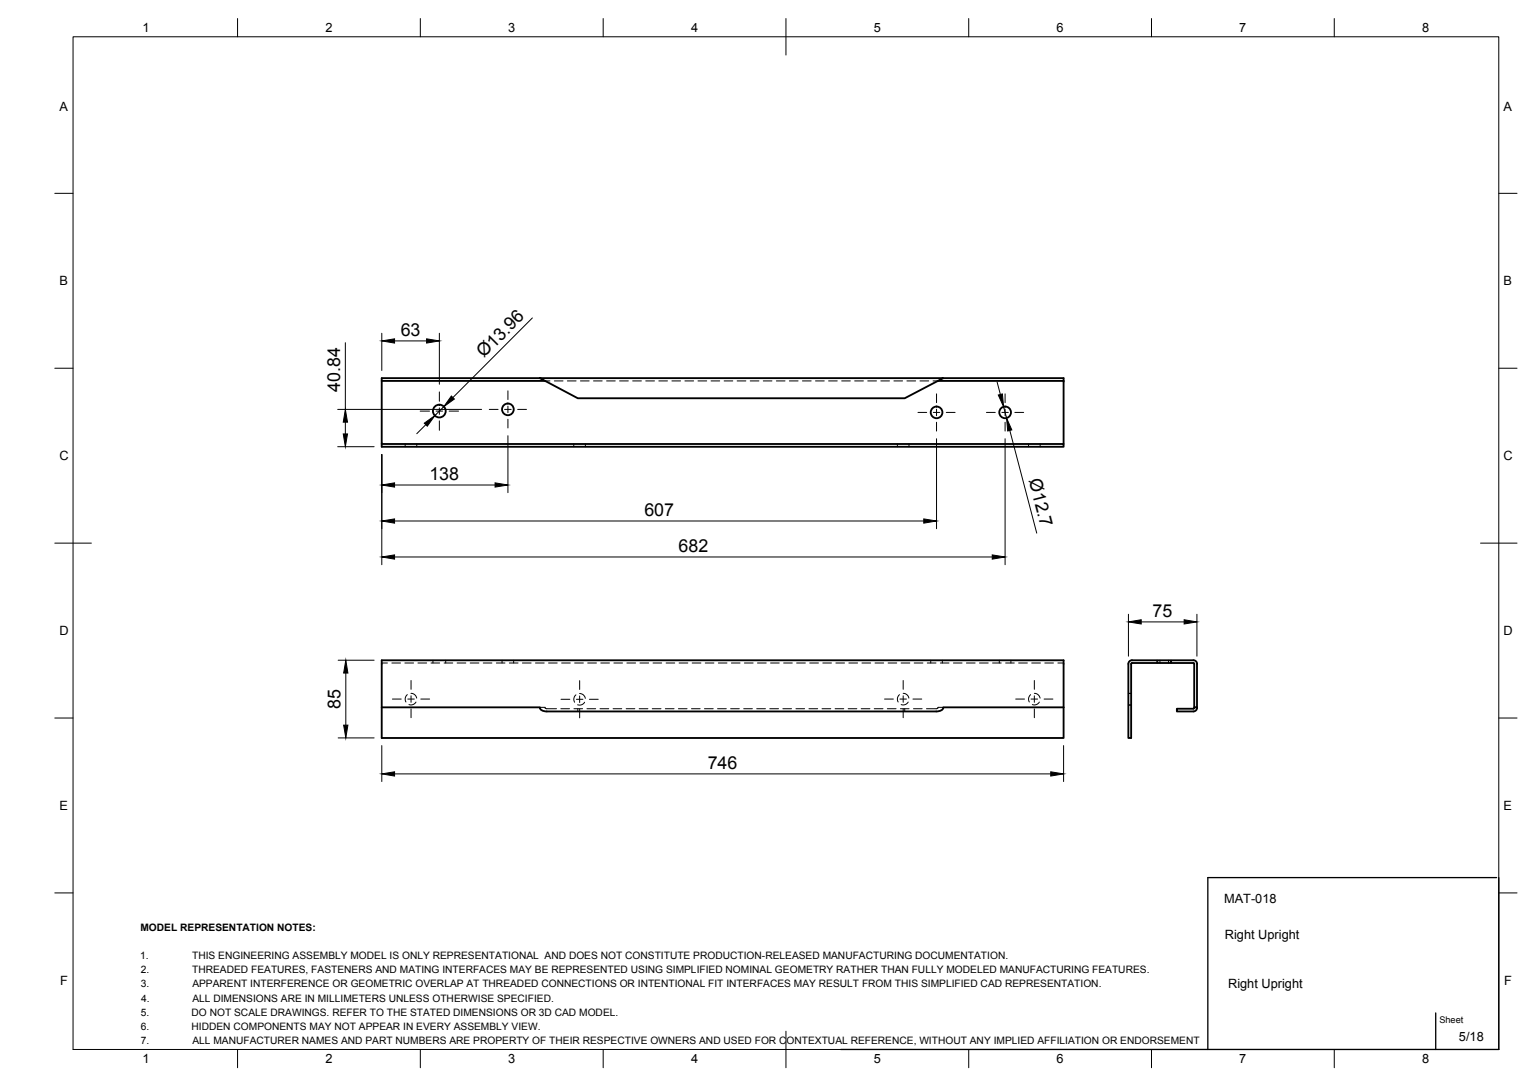
ISO-10303-21;
HEADER;
/* Generated by software containing ST-Developer
 * from STEP Tools, Inc. (www.steptools.com) 
 */

FILE_DESCRIPTION(
/* description */ ('STEP AP214'),
/* implementation_level */ '2;1');

FILE_NAME(
/* name */ 'Right Upright.step',
/* time_stamp */ '2026-11-14T06:16:09-08:00',
/* author */ (''),
/* organization */ (''),
/* preprocessor_version */ 'ST-DEVELOPER v20.2',
/* originating_system */ 'Autodesk Translation Framework v15.17.0.0',
/* authorisation */ '');

FILE_SCHEMA (('AUTOMOTIVE_DESIGN { 1 0 10303 214 3 1 1 }'));
ENDSEC;

DATA;
#10=MECHANICAL_DESIGN_GEOMETRIC_PRESENTATION_REPRESENTATION('',(#349),#18006);
#268=ELLIPSE('',#10059,8.64513309637285,4.00000000000059);
#269=ELLIPSE('',#10060,8.53586336233429,3.99999999999978);
#270=ELLIPSE('',#10073,2.16128327409315,1.00000000000008);
#271=ELLIPSE('',#10074,2.1339658405822,0.999999999999361);
#317=SHAPE_REPRESENTATION_RELATIONSHIP('SRR','None',#18073,#333);
#333=ADVANCED_BREP_SHAPE_REPRESENTATION('',(#365),#17990);
#349=STYLED_ITEM('',(#18170),#365);
#365=MANIFOLD_SOLID_BREP('Body1',#9558);
#417=FACE_BOUND('',#1638,.T.);
#418=FACE_BOUND('',#1639,.T.);
#419=FACE_BOUND('',#1640,.T.);
#420=FACE_BOUND('',#1641,.T.);
#421=FACE_BOUND('',#1644,.T.);
#422=FACE_BOUND('',#1645,.T.);
#423=FACE_BOUND('',#1646,.T.);
#424=FACE_BOUND('',#1647,.T.);
#425=FACE_BOUND('',#1650,.T.);
#426=FACE_BOUND('',#1651,.T.);
#427=FACE_BOUND('',#1652,.T.);
#428=FACE_BOUND('',#1653,.T.);
#429=FACE_BOUND('',#1656,.T.);
#430=FACE_BOUND('',#1657,.T.);
#431=FACE_BOUND('',#1658,.T.);
#432=FACE_BOUND('',#1659,.T.);
#614=PLANE('',#10038);
#615=PLANE('',#10039);
#616=PLANE('',#10042);
#617=PLANE('',#10043);
#618=PLANE('',#10046);
#619=PLANE('',#10047);
#620=PLANE('',#10050);
#621=PLANE('',#10051);
#622=PLANE('',#10054);
#623=PLANE('',#10055);
#624=PLANE('',#10056);
#625=PLANE('',#10057);
#626=PLANE('',#10061);
#627=PLANE('',#10063);
#628=PLANE('',#10065);
#629=PLANE('',#10066);
#630=PLANE('',#10067);
#631=PLANE('',#10069);
#632=PLANE('',#10071);
#633=PLANE('',#10075);
#634=PLANE('',#10076);
#635=PLANE('',#10077);
#636=PLANE('',#10078);
#637=PLANE('',#10079);
#1000=FACE_OUTER_BOUND('',#1614,.T.);
#1001=FACE_OUTER_BOUND('',#1615,.T.);
#1002=FACE_OUTER_BOUND('',#1616,.T.);
#1003=FACE_OUTER_BOUND('',#1617,.T.);
#1004=FACE_OUTER_BOUND('',#1618,.T.);
#1005=FACE_OUTER_BOUND('',#1619,.T.);
#1006=FACE_OUTER_BOUND('',#1620,.T.);
#1007=FACE_OUTER_BOUND('',#1621,.T.);
#1008=FACE_OUTER_BOUND('',#1622,.T.);
#1009=FACE_OUTER_BOUND('',#1623,.T.);
#1010=FACE_OUTER_BOUND('',#1624,.T.);
#1011=FACE_OUTER_BOUND('',#1625,.T.);
#1012=FACE_OUTER_BOUND('',#1626,.T.);
#1013=FACE_OUTER_BOUND('',#1627,.T.);
#1014=FACE_OUTER_BOUND('',#1628,.T.);
#1015=FACE_OUTER_BOUND('',#1629,.T.);
#1016=FACE_OUTER_BOUND('',#1630,.T.);
#1017=FACE_OUTER_BOUND('',#1631,.T.);
#1018=FACE_OUTER_BOUND('',#1632,.T.);
#1019=FACE_OUTER_BOUND('',#1633,.T.);
#1020=FACE_OUTER_BOUND('',#1634,.T.);
#1021=FACE_OUTER_BOUND('',#1635,.T.);
#1022=FACE_OUTER_BOUND('',#1636,.T.);
#1023=FACE_OUTER_BOUND('',#1637,.T.);
#1024=FACE_OUTER_BOUND('',#1642,.T.);
#1025=FACE_OUTER_BOUND('',#1643,.T.);
#1026=FACE_OUTER_BOUND('',#1648,.T.);
#1027=FACE_OUTER_BOUND('',#1649,.T.);
#1028=FACE_OUTER_BOUND('',#1654,.T.);
#1029=FACE_OUTER_BOUND('',#1655,.T.);
#1030=FACE_OUTER_BOUND('',#1660,.T.);
#1031=FACE_OUTER_BOUND('',#1661,.T.);
#1032=FACE_OUTER_BOUND('',#1662,.T.);
#1033=FACE_OUTER_BOUND('',#1663,.T.);
#1034=FACE_OUTER_BOUND('',#1664,.T.);
#1035=FACE_OUTER_BOUND('',#1665,.T.);
#1036=FACE_OUTER_BOUND('',#1666,.T.);
#1037=FACE_OUTER_BOUND('',#1667,.T.);
#1614=EDGE_LOOP('',(#6874,#6875,#6876,#6877));
#1615=EDGE_LOOP('',(#6878,#6879,#6880,#6881));
#1616=EDGE_LOOP('',(#6882,#6883,#6884,#6885));
#1617=EDGE_LOOP('',(#6886,#6887,#6888,#6889));
#1618=EDGE_LOOP('',(#6890,#6891,#6892,#6893));
#1619=EDGE_LOOP('',(#6894,#6895,#6896,#6897));
#1620=EDGE_LOOP('',(#6898,#6899,#6900,#6901));
#1621=EDGE_LOOP('',(#6902,#6903,#6904,#6905));
#1622=EDGE_LOOP('',(#6906,#6907,#6908,#6909));
#1623=EDGE_LOOP('',(#6910,#6911,#6912,#6913));
#1624=EDGE_LOOP('',(#6914,#6915,#6916,#6917));
#1625=EDGE_LOOP('',(#6918,#6919,#6920,#6921));
#1626=EDGE_LOOP('',(#6922,#6923,#6924,#6925));
#1627=EDGE_LOOP('',(#6926,#6927,#6928,#6929));
#1628=EDGE_LOOP('',(#6930,#6931,#6932,#6933));
#1629=EDGE_LOOP('',(#6934,#6935,#6936,#6937));
#1630=EDGE_LOOP('',(#6938,#6939,#6940,#6941));
#1631=EDGE_LOOP('',(#6942,#6943,#6944,#6945));
#1632=EDGE_LOOP('',(#6946,#6947,#6948,#6949));
#1633=EDGE_LOOP('',(#6950,#6951,#6952,#6953));
#1634=EDGE_LOOP('',(#6954,#6955,#6956,#6957));
#1635=EDGE_LOOP('',(#6958,#6959,#6960,#6961,#6962,#6963,#6964,#6965));
#1636=EDGE_LOOP('',(#6966,#6967,#6968,#6969));
#1637=EDGE_LOOP('',(#6970,#6971,#6972,#6973));
#1638=EDGE_LOOP('',(#6974));
#1639=EDGE_LOOP('',(#6975));
#1640=EDGE_LOOP('',(#6976));
#1641=EDGE_LOOP('',(#6977));
#1642=EDGE_LOOP('',(#6978,#6979,#6980,#6981));
#1643=EDGE_LOOP('',(#6982,#6983,#6984,#6985));
#1644=EDGE_LOOP('',(#6986));
#1645=EDGE_LOOP('',(#6987));
#1646=EDGE_LOOP('',(#6988));
#1647=EDGE_LOOP('',(#6989));
#1648=EDGE_LOOP('',(#6990,#6991,#6992,#6993));
#1649=EDGE_LOOP('',(#6994,#6995,#6996,#6997));
#1650=EDGE_LOOP('',(#6998));
#1651=EDGE_LOOP('',(#6999));
#1652=EDGE_LOOP('',(#7000));
#1653=EDGE_LOOP('',(#7001));
#1654=EDGE_LOOP('',(#7002,#7003,#7004,#7005));
#1655=EDGE_LOOP('',(#7006,#7007,#7008,#7009));
#1656=EDGE_LOOP('',(#7010));
#1657=EDGE_LOOP('',(#7011));
#1658=EDGE_LOOP('',(#7012));
#1659=EDGE_LOOP('',(#7013));
#1660=EDGE_LOOP('',(#7014,#7015,#7016,#7017));
#1661=EDGE_LOOP('',(#7018,#7019,#7020,#7021,#7022,#7023,#7024,#7025));
#1662=EDGE_LOOP('',(#7026,#7027,#7028,#7029));
#1663=EDGE_LOOP('',(#7030,#7031,#7032,#7033));
#1664=EDGE_LOOP('',(#7034,#7035,#7036,#7037));
#1665=EDGE_LOOP('',(#7038,#7039,#7040,#7041,#7042,#7043,#7044,#7045));
#1666=EDGE_LOOP('',(#7046,#7047,#7048,#7049,#7050,#7051,#7052,#7053));
#1667=EDGE_LOOP('',(#7054,#7055,#7056,#7057));
#2375=LINE('',#14543,#3099);
#2376=LINE('',#14549,#3100);
#2377=LINE('',#14555,#3101);
#2378=LINE('',#14561,#3102);
#2379=LINE('',#14567,#3103);
#2380=LINE('',#14573,#3104);
#2381=LINE('',#14579,#3105);
#2382=LINE('',#14585,#3106);
#2383=LINE('',#14590,#3107);
#2384=LINE('',#14592,#3108);
#2385=LINE('',#14594,#3109);
#2386=LINE('',#14595,#3110);
#2387=LINE('',#14599,#3111);
#2388=LINE('',#14603,#3112);
#2389=LINE('',#14607,#3113);
#2390=LINE('',#14609,#3114);
#2391=LINE('',#14610,#3115);
#2392=LINE('',#14614,#3116);
#2393=LINE('',#14618,#3117);
#2394=LINE('',#14622,#3118);
#2395=LINE('',#14624,#3119);
#2396=LINE('',#14625,#3120);
#2397=LINE('',#14629,#3121);
#2398=LINE('',#14633,#3122);
#2399=LINE('',#14636,#3123);
#2400=LINE('',#14637,#3124);
#2401=LINE('',#14644,#3125);
#2402=LINE('',#14645,#3126);
#2403=LINE('',#14646,#3127);
#2404=LINE('',#14650,#3128);
#2405=LINE('',#14652,#3129);
#2406=LINE('',#14654,#3130);
#2407=LINE('',#14655,#3131);
#2408=LINE('',#14658,#3132);
#2409=LINE('',#14660,#3133);
#2410=LINE('',#14661,#3134);
#2411=LINE('',#14664,#3135);
#2412=LINE('',#14666,#3136);
#2413=LINE('',#14667,#3137);
#2414=LINE('',#14672,#3138);
#2415=LINE('',#14676,#3139);
#2416=LINE('',#14677,#3140);
#2417=LINE('',#14678,#3141);
#2418=LINE('',#14680,#3142);
#2419=LINE('',#14681,#3143);
#2420=LINE('',#14683,#3144);
#2421=LINE('',#14685,#3145);
#2422=LINE('',#14687,#3146);
#2423=LINE('',#14690,#3147);
#2424=LINE('',#14691,#3148);
#2425=LINE('',#14694,#3149);
#2426=LINE('',#14695,#3150);
#2427=LINE('',#14697,#3151);
#2428=LINE('',#14698,#3152);
#2429=LINE('',#14700,#3153);
#2430=LINE('',#14702,#3154);
#2431=LINE('',#14704,#3155);
#2432=LINE('',#14707,#3156);
#2433=LINE('',#14709,#3157);
#2434=LINE('',#14711,#3158);
#2435=LINE('',#14713,#3159);
#2436=LINE('',#14714,#3160);
#2437=LINE('',#14720,#3161);
#2438=LINE('',#14723,#3162);
#3099=VECTOR('',#11654,6.34999999871023);
#3100=VECTOR('',#11661,6.34999999871025);
#3101=VECTOR('',#11668,6.34999999999997);
#3102=VECTOR('',#11675,6.98053323984749);
#3103=VECTOR('',#11682,6.35);
#3104=VECTOR('',#11689,6.34999999999999);
#3105=VECTOR('',#11696,6.35);
#3106=VECTOR('',#11703,6.35);
#3107=VECTOR('',#11708,1000.);
#3108=VECTOR('',#11709,1000.);
#3109=VECTOR('',#11710,1000.);
#3110=VECTOR('',#11711,1000.);
#3111=VECTOR('',#11714,1000.);
#3112=VECTOR('',#11717,1000.);
#3113=VECTOR('',#11722,1000.);
#3114=VECTOR('',#11723,1000.);
#3115=VECTOR('',#11724,1000.);
#3116=VECTOR('',#11727,1000.);
#3117=VECTOR('',#11730,1000.);
#3118=VECTOR('',#11735,1000.);
#3119=VECTOR('',#11736,1000.);
#3120=VECTOR('',#11737,1000.);
#3121=VECTOR('',#11740,1000.);
#3122=VECTOR('',#11743,1000.);
#3123=VECTOR('',#11748,1000.);
#3124=VECTOR('',#11749,1000.);
#3125=VECTOR('',#11758,1000.);
#3126=VECTOR('',#11759,1000.);
#3127=VECTOR('',#11760,1000.);
#3128=VECTOR('',#11763,1000.);
#3129=VECTOR('',#11764,1000.);
#3130=VECTOR('',#11765,1000.);
#3131=VECTOR('',#11766,1000.);
#3132=VECTOR('',#11769,1000.);
#3133=VECTOR('',#11770,1000.);
#3134=VECTOR('',#11771,1000.);
#3135=VECTOR('',#11774,1000.);
#3136=VECTOR('',#11775,1000.);
#3137=VECTOR('',#11776,1000.);
#3138=VECTOR('',#11781,1000.);
#3139=VECTOR('',#11786,1000.);
#3140=VECTOR('',#11787,1000.);
#3141=VECTOR('',#11788,1000.);
#3142=VECTOR('',#11789,1000.);
#3143=VECTOR('',#11790,1000.);
#3144=VECTOR('',#11793,1000.);
#3145=VECTOR('',#11796,1000.);
#3146=VECTOR('',#11799,1000.);
#3147=VECTOR('',#11802,1000.);
#3148=VECTOR('',#11803,1000.);
#3149=VECTOR('',#11806,1000.);
#3150=VECTOR('',#11807,1000.);
#3151=VECTOR('',#11810,1000.);
#3152=VECTOR('',#11811,1000.);
#3153=VECTOR('',#11814,1000.);
#3154=VECTOR('',#11817,1000.);
#3155=VECTOR('',#11820,1000.);
#3156=VECTOR('',#11823,1000.);
#3157=VECTOR('',#11824,1000.);
#3158=VECTOR('',#11825,1000.);
#3159=VECTOR('',#11826,1000.);
#3160=VECTOR('',#11827,1000.);
#3161=VECTOR('',#11838,1000.);
#3162=VECTOR('',#11843,1000.);
#3666=CIRCLE('',#10015,6.34999999871023);
#3667=CIRCLE('',#10016,6.34999999871023);
#3668=CIRCLE('',#10018,6.34999999871025);
#3669=CIRCLE('',#10019,6.34999999871025);
#3670=CIRCLE('',#10021,6.34999999999997);
#3671=CIRCLE('',#10022,6.34999999999997);
#3672=CIRCLE('',#10024,6.98053323984749);
#3673=CIRCLE('',#10025,6.98053323984749);
#3674=CIRCLE('',#10027,6.35);
#3675=CIRCLE('',#10028,6.35);
#3676=CIRCLE('',#10030,6.34999999999999);
#3677=CIRCLE('',#10031,6.34999999999999);
#3678=CIRCLE('',#10033,6.35);
#3679=CIRCLE('',#10034,6.35);
#3680=CIRCLE('',#10036,6.35);
#3681=CIRCLE('',#10037,6.35);
#3682=CIRCLE('',#10040,1.);
#3683=CIRCLE('',#10041,4.);
#3684=CIRCLE('',#10044,1.);
#3685=CIRCLE('',#10045,4.);
#3686=CIRCLE('',#10048,1.);
#3687=CIRCLE('',#10049,4.);
#3688=CIRCLE('',#10052,1.);
#3689=CIRCLE('',#10053,4.);
#4219=VERTEX_POINT('',#14540);
#4220=VERTEX_POINT('',#14542);
#4221=VERTEX_POINT('',#14546);
#4222=VERTEX_POINT('',#14548);
#4223=VERTEX_POINT('',#14552);
#4224=VERTEX_POINT('',#14554);
#4225=VERTEX_POINT('',#14558);
#4226=VERTEX_POINT('',#14560);
#4227=VERTEX_POINT('',#14564);
#4228=VERTEX_POINT('',#14566);
#4229=VERTEX_POINT('',#14570);
#4230=VERTEX_POINT('',#14572);
#4231=VERTEX_POINT('',#14576);
#4232=VERTEX_POINT('',#14578);
#4233=VERTEX_POINT('',#14582);
#4234=VERTEX_POINT('',#14584);
#4235=VERTEX_POINT('',#14588);
#4236=VERTEX_POINT('',#14589);
#4237=VERTEX_POINT('',#14591);
#4238=VERTEX_POINT('',#14593);
#4239=VERTEX_POINT('',#14597);
#4240=VERTEX_POINT('',#14598);
#4241=VERTEX_POINT('',#14600);
#4242=VERTEX_POINT('',#14602);
#4243=VERTEX_POINT('',#14606);
#4244=VERTEX_POINT('',#14608);
#4245=VERTEX_POINT('',#14612);
#4246=VERTEX_POINT('',#14613);
#4247=VERTEX_POINT('',#14615);
#4248=VERTEX_POINT('',#14617);
#4249=VERTEX_POINT('',#14621);
#4250=VERTEX_POINT('',#14623);
#4251=VERTEX_POINT('',#14627);
#4252=VERTEX_POINT('',#14628);
#4253=VERTEX_POINT('',#14630);
#4254=VERTEX_POINT('',#14632);
#4255=VERTEX_POINT('',#14642);
#4256=VERTEX_POINT('',#14643);
#4257=VERTEX_POINT('',#14648);
#4258=VERTEX_POINT('',#14649);
#4259=VERTEX_POINT('',#14651);
#4260=VERTEX_POINT('',#14653);
#4261=VERTEX_POINT('',#14657);
#4262=VERTEX_POINT('',#14659);
#4263=VERTEX_POINT('',#14663);
#4264=VERTEX_POINT('',#14665);
#4265=VERTEX_POINT('',#14669);
#4266=VERTEX_POINT('',#14671);
#4267=VERTEX_POINT('',#14675);
#4268=VERTEX_POINT('',#14679);
#4269=VERTEX_POINT('',#14689);
#4270=VERTEX_POINT('',#14693);
#4271=VERTEX_POINT('',#14706);
#4272=VERTEX_POINT('',#14708);
#4273=VERTEX_POINT('',#14710);
#4274=VERTEX_POINT('',#14712);
#5185=EDGE_CURVE('',#4219,#4219,#3666,.T.);
#5186=EDGE_CURVE('',#4219,#4220,#2375,.T.);
#5187=EDGE_CURVE('',#4220,#4220,#3667,.T.);
#5188=EDGE_CURVE('',#4221,#4221,#3668,.T.);
#5189=EDGE_CURVE('',#4221,#4222,#2376,.T.);
#5190=EDGE_CURVE('',#4222,#4222,#3669,.T.);
#5191=EDGE_CURVE('',#4223,#4223,#3670,.T.);
#5192=EDGE_CURVE('',#4223,#4224,#2377,.T.);
#5193=EDGE_CURVE('',#4224,#4224,#3671,.T.);
#5194=EDGE_CURVE('',#4225,#4225,#3672,.T.);
#5195=EDGE_CURVE('',#4225,#4226,#2378,.T.);
#5196=EDGE_CURVE('',#4226,#4226,#3673,.T.);
#5197=EDGE_CURVE('',#4227,#4227,#3674,.T.);
#5198=EDGE_CURVE('',#4227,#4228,#2379,.T.);
#5199=EDGE_CURVE('',#4228,#4228,#3675,.T.);
#5200=EDGE_CURVE('',#4229,#4229,#3676,.T.);
#5201=EDGE_CURVE('',#4229,#4230,#2380,.T.);
#5202=EDGE_CURVE('',#4230,#4230,#3677,.T.);
#5203=EDGE_CURVE('',#4231,#4231,#3678,.T.);
#5204=EDGE_CURVE('',#4231,#4232,#2381,.T.);
#5205=EDGE_CURVE('',#4232,#4232,#3679,.T.);
#5206=EDGE_CURVE('',#4233,#4233,#3680,.T.);
#5207=EDGE_CURVE('',#4233,#4234,#2382,.T.);
#5208=EDGE_CURVE('',#4234,#4234,#3681,.T.);
#5209=EDGE_CURVE('',#4235,#4236,#2383,.T.);
#5210=EDGE_CURVE('',#4236,#4237,#2384,.T.);
#5211=EDGE_CURVE('',#4238,#4237,#2385,.T.);
#5212=EDGE_CURVE('',#4238,#4235,#2386,.T.);
#5213=EDGE_CURVE('',#4239,#4240,#2387,.T.);
#5214=EDGE_CURVE('',#4239,#4241,#3682,.T.);
#5215=EDGE_CURVE('',#4242,#4241,#2388,.T.);
#5216=EDGE_CURVE('',#4240,#4242,#3683,.T.);
#5217=EDGE_CURVE('',#4243,#4239,#2389,.T.);
#5218=EDGE_CURVE('',#4244,#4240,#2390,.T.);
#5219=EDGE_CURVE('',#4243,#4244,#2391,.T.);
#5220=EDGE_CURVE('',#4245,#4246,#2392,.T.);
#5221=EDGE_CURVE('',#4247,#4245,#3684,.T.);
#5222=EDGE_CURVE('',#4248,#4247,#2393,.T.);
#5223=EDGE_CURVE('',#4248,#4246,#3685,.T.);
#5224=EDGE_CURVE('',#4245,#4249,#2394,.T.);
#5225=EDGE_CURVE('',#4246,#4250,#2395,.T.);
#5226=EDGE_CURVE('',#4250,#4249,#2396,.T.);
#5227=EDGE_CURVE('',#4251,#4252,#2397,.T.);
#5228=EDGE_CURVE('',#4251,#4253,#3686,.T.);
#5229=EDGE_CURVE('',#4254,#4253,#2398,.T.);
#5230=EDGE_CURVE('',#4252,#4254,#3687,.T.);
#5231=EDGE_CURVE('',#4241,#4251,#2399,.T.);
#5232=EDGE_CURVE('',#4242,#4252,#2400,.T.);
#5233=EDGE_CURVE('',#4249,#4238,#3688,.T.);
#5234=EDGE_CURVE('',#4250,#4235,#3689,.T.);
#5235=EDGE_CURVE('',#4255,#4256,#2401,.T.);
#5236=EDGE_CURVE('',#4254,#4255,#2402,.T.);
#5237=EDGE_CURVE('',#4253,#4256,#2403,.T.);
#5238=EDGE_CURVE('',#4257,#4258,#2404,.T.);
#5239=EDGE_CURVE('',#4258,#4259,#2405,.T.);
#5240=EDGE_CURVE('',#4260,#4259,#2406,.T.);
#5241=EDGE_CURVE('',#4260,#4257,#2407,.T.);
#5242=EDGE_CURVE('',#4259,#4261,#2408,.T.);
#5243=EDGE_CURVE('',#4262,#4261,#2409,.T.);
#5244=EDGE_CURVE('',#4260,#4262,#2410,.T.);
#5245=EDGE_CURVE('',#4263,#4261,#2411,.T.);
#5246=EDGE_CURVE('',#4264,#4263,#2412,.T.);
#5247=EDGE_CURVE('',#4262,#4264,#2413,.T.);
#5248=EDGE_CURVE('',#4265,#4263,#268,.T.);
#5249=EDGE_CURVE('',#4266,#4265,#2414,.T.);
#5250=EDGE_CURVE('',#4264,#4266,#269,.T.);
#5251=EDGE_CURVE('',#4267,#4265,#2415,.T.);
#5252=EDGE_CURVE('',#4267,#4236,#2416,.T.);
#5253=EDGE_CURVE('',#4254,#4235,#2417,.T.);
#5254=EDGE_CURVE('',#4268,#4255,#2418,.T.);
#5255=EDGE_CURVE('',#4266,#4268,#2419,.T.);
#5256=EDGE_CURVE('',#4252,#4250,#2420,.T.);
#5257=EDGE_CURVE('',#4242,#4246,#2421,.T.);
#5258=EDGE_CURVE('',#4240,#4248,#2422,.T.);
#5259=EDGE_CURVE('',#4269,#4248,#2423,.T.);
#5260=EDGE_CURVE('',#4244,#4269,#2424,.T.);
#5261=EDGE_CURVE('',#4270,#4269,#2425,.T.);
#5262=EDGE_CURVE('',#4243,#4270,#2426,.T.);
#5263=EDGE_CURVE('',#4270,#4247,#2427,.T.);
#5264=EDGE_CURVE('',#4239,#4247,#2428,.T.);
#5265=EDGE_CURVE('',#4241,#4245,#2429,.T.);
#5266=EDGE_CURVE('',#4251,#4249,#2430,.T.);
#5267=EDGE_CURVE('',#4253,#4238,#2431,.T.);
#5268=EDGE_CURVE('',#4271,#4237,#2432,.T.);
#5269=EDGE_CURVE('',#4271,#4272,#2433,.T.);
#5270=EDGE_CURVE('',#4273,#4272,#2434,.T.);
#5271=EDGE_CURVE('',#4273,#4274,#2435,.T.);
#5272=EDGE_CURVE('',#4274,#4256,#2436,.T.);
#5273=EDGE_CURVE('',#4272,#4258,#270,.T.);
#5274=EDGE_CURVE('',#4257,#4273,#271,.T.);
#5275=EDGE_CURVE('',#4274,#4268,#2437,.T.);
#5276=EDGE_CURVE('',#4267,#4271,#2438,.T.);
#6874=ORIENTED_EDGE('',*,*,#5185,.F.);
#6875=ORIENTED_EDGE('',*,*,#5186,.T.);
#6876=ORIENTED_EDGE('',*,*,#5187,.T.);
#6877=ORIENTED_EDGE('',*,*,#5186,.F.);
#6878=ORIENTED_EDGE('',*,*,#5188,.F.);
#6879=ORIENTED_EDGE('',*,*,#5189,.T.);
#6880=ORIENTED_EDGE('',*,*,#5190,.T.);
#6881=ORIENTED_EDGE('',*,*,#5189,.F.);
#6882=ORIENTED_EDGE('',*,*,#5191,.F.);
#6883=ORIENTED_EDGE('',*,*,#5192,.T.);
#6884=ORIENTED_EDGE('',*,*,#5193,.T.);
#6885=ORIENTED_EDGE('',*,*,#5192,.F.);
#6886=ORIENTED_EDGE('',*,*,#5194,.F.);
#6887=ORIENTED_EDGE('',*,*,#5195,.T.);
#6888=ORIENTED_EDGE('',*,*,#5196,.T.);
#6889=ORIENTED_EDGE('',*,*,#5195,.F.);
#6890=ORIENTED_EDGE('',*,*,#5197,.F.);
#6891=ORIENTED_EDGE('',*,*,#5198,.T.);
#6892=ORIENTED_EDGE('',*,*,#5199,.T.);
#6893=ORIENTED_EDGE('',*,*,#5198,.F.);
#6894=ORIENTED_EDGE('',*,*,#5200,.F.);
#6895=ORIENTED_EDGE('',*,*,#5201,.T.);
#6896=ORIENTED_EDGE('',*,*,#5202,.T.);
#6897=ORIENTED_EDGE('',*,*,#5201,.F.);
#6898=ORIENTED_EDGE('',*,*,#5203,.F.);
#6899=ORIENTED_EDGE('',*,*,#5204,.T.);
#6900=ORIENTED_EDGE('',*,*,#5205,.T.);
#6901=ORIENTED_EDGE('',*,*,#5204,.F.);
#6902=ORIENTED_EDGE('',*,*,#5206,.F.);
#6903=ORIENTED_EDGE('',*,*,#5207,.T.);
#6904=ORIENTED_EDGE('',*,*,#5208,.T.);
#6905=ORIENTED_EDGE('',*,*,#5207,.F.);
#6906=ORIENTED_EDGE('',*,*,#5209,.T.);
#6907=ORIENTED_EDGE('',*,*,#5210,.T.);
#6908=ORIENTED_EDGE('',*,*,#5211,.F.);
#6909=ORIENTED_EDGE('',*,*,#5212,.T.);
#6910=ORIENTED_EDGE('',*,*,#5213,.F.);
#6911=ORIENTED_EDGE('',*,*,#5214,.T.);
#6912=ORIENTED_EDGE('',*,*,#5215,.F.);
#6913=ORIENTED_EDGE('',*,*,#5216,.F.);
#6914=ORIENTED_EDGE('',*,*,#5217,.T.);
#6915=ORIENTED_EDGE('',*,*,#5213,.T.);
#6916=ORIENTED_EDGE('',*,*,#5218,.F.);
#6917=ORIENTED_EDGE('',*,*,#5219,.F.);
#6918=ORIENTED_EDGE('',*,*,#5220,.F.);
#6919=ORIENTED_EDGE('',*,*,#5221,.F.);
#6920=ORIENTED_EDGE('',*,*,#5222,.F.);
#6921=ORIENTED_EDGE('',*,*,#5223,.T.);
#6922=ORIENTED_EDGE('',*,*,#5224,.F.);
#6923=ORIENTED_EDGE('',*,*,#5220,.T.);
#6924=ORIENTED_EDGE('',*,*,#5225,.T.);
#6925=ORIENTED_EDGE('',*,*,#5226,.T.);
#6926=ORIENTED_EDGE('',*,*,#5227,.F.);
#6927=ORIENTED_EDGE('',*,*,#5228,.T.);
#6928=ORIENTED_EDGE('',*,*,#5229,.F.);
#6929=ORIENTED_EDGE('',*,*,#5230,.F.);
#6930=ORIENTED_EDGE('',*,*,#5231,.T.);
#6931=ORIENTED_EDGE('',*,*,#5227,.T.);
#6932=ORIENTED_EDGE('',*,*,#5232,.F.);
#6933=ORIENTED_EDGE('',*,*,#5215,.T.);
#6934=ORIENTED_EDGE('',*,*,#5212,.F.);
#6935=ORIENTED_EDGE('',*,*,#5233,.F.);
#6936=ORIENTED_EDGE('',*,*,#5226,.F.);
#6937=ORIENTED_EDGE('',*,*,#5234,.T.);
#6938=ORIENTED_EDGE('',*,*,#5235,.F.);
#6939=ORIENTED_EDGE('',*,*,#5236,.F.);
#6940=ORIENTED_EDGE('',*,*,#5229,.T.);
#6941=ORIENTED_EDGE('',*,*,#5237,.T.);
#6942=ORIENTED_EDGE('',*,*,#5238,.T.);
#6943=ORIENTED_EDGE('',*,*,#5239,.T.);
#6944=ORIENTED_EDGE('',*,*,#5240,.F.);
#6945=ORIENTED_EDGE('',*,*,#5241,.T.);
#6946=ORIENTED_EDGE('',*,*,#5242,.T.);
#6947=ORIENTED_EDGE('',*,*,#5243,.F.);
#6948=ORIENTED_EDGE('',*,*,#5244,.F.);
#6949=ORIENTED_EDGE('',*,*,#5240,.T.);
#6950=ORIENTED_EDGE('',*,*,#5245,.F.);
#6951=ORIENTED_EDGE('',*,*,#5246,.F.);
#6952=ORIENTED_EDGE('',*,*,#5247,.F.);
#6953=ORIENTED_EDGE('',*,*,#5243,.T.);
#6954=ORIENTED_EDGE('',*,*,#5248,.F.);
#6955=ORIENTED_EDGE('',*,*,#5249,.F.);
#6956=ORIENTED_EDGE('',*,*,#5250,.F.);
#6957=ORIENTED_EDGE('',*,*,#5246,.T.);
#6958=ORIENTED_EDGE('',*,*,#5251,.F.);
#6959=ORIENTED_EDGE('',*,*,#5252,.T.);
#6960=ORIENTED_EDGE('',*,*,#5209,.F.);
#6961=ORIENTED_EDGE('',*,*,#5253,.F.);
#6962=ORIENTED_EDGE('',*,*,#5236,.T.);
#6963=ORIENTED_EDGE('',*,*,#5254,.F.);
#6964=ORIENTED_EDGE('',*,*,#5255,.F.);
#6965=ORIENTED_EDGE('',*,*,#5249,.T.);
#6966=ORIENTED_EDGE('',*,*,#5234,.F.);
#6967=ORIENTED_EDGE('',*,*,#5256,.F.);
#6968=ORIENTED_EDGE('',*,*,#5230,.T.);
#6969=ORIENTED_EDGE('',*,*,#5253,.T.);
#6970=ORIENTED_EDGE('',*,*,#5225,.F.);
#6971=ORIENTED_EDGE('',*,*,#5257,.F.);
#6972=ORIENTED_EDGE('',*,*,#5232,.T.);
#6973=ORIENTED_EDGE('',*,*,#5256,.T.);
#6974=ORIENTED_EDGE('',*,*,#5187,.F.);
#6975=ORIENTED_EDGE('',*,*,#5190,.F.);
#6976=ORIENTED_EDGE('',*,*,#5193,.F.);
#6977=ORIENTED_EDGE('',*,*,#5196,.F.);
#6978=ORIENTED_EDGE('',*,*,#5223,.F.);
#6979=ORIENTED_EDGE('',*,*,#5258,.F.);
#6980=ORIENTED_EDGE('',*,*,#5216,.T.);
#6981=ORIENTED_EDGE('',*,*,#5257,.T.);
#6982=ORIENTED_EDGE('',*,*,#5259,.F.);
#6983=ORIENTED_EDGE('',*,*,#5260,.F.);
#6984=ORIENTED_EDGE('',*,*,#5218,.T.);
#6985=ORIENTED_EDGE('',*,*,#5258,.T.);
#6986=ORIENTED_EDGE('',*,*,#5199,.F.);
#6987=ORIENTED_EDGE('',*,*,#5202,.F.);
#6988=ORIENTED_EDGE('',*,*,#5205,.F.);
#6989=ORIENTED_EDGE('',*,*,#5208,.F.);
#6990=ORIENTED_EDGE('',*,*,#5261,.F.);
#6991=ORIENTED_EDGE('',*,*,#5262,.F.);
#6992=ORIENTED_EDGE('',*,*,#5219,.T.);
#6993=ORIENTED_EDGE('',*,*,#5260,.T.);
#6994=ORIENTED_EDGE('',*,*,#5263,.T.);
#6995=ORIENTED_EDGE('',*,*,#5264,.F.);
#6996=ORIENTED_EDGE('',*,*,#5217,.F.);
#6997=ORIENTED_EDGE('',*,*,#5262,.T.);
#6998=ORIENTED_EDGE('',*,*,#5197,.T.);
#6999=ORIENTED_EDGE('',*,*,#5200,.T.);
#7000=ORIENTED_EDGE('',*,*,#5203,.T.);
#7001=ORIENTED_EDGE('',*,*,#5206,.T.);
#7002=ORIENTED_EDGE('',*,*,#5221,.T.);
#7003=ORIENTED_EDGE('',*,*,#5265,.F.);
#7004=ORIENTED_EDGE('',*,*,#5214,.F.);
#7005=ORIENTED_EDGE('',*,*,#5264,.T.);
#7006=ORIENTED_EDGE('',*,*,#5224,.T.);
#7007=ORIENTED_EDGE('',*,*,#5266,.F.);
#7008=ORIENTED_EDGE('',*,*,#5231,.F.);
#7009=ORIENTED_EDGE('',*,*,#5265,.T.);
#7010=ORIENTED_EDGE('',*,*,#5185,.T.);
#7011=ORIENTED_EDGE('',*,*,#5188,.T.);
#7012=ORIENTED_EDGE('',*,*,#5191,.T.);
#7013=ORIENTED_EDGE('',*,*,#5194,.T.);
#7014=ORIENTED_EDGE('',*,*,#5233,.T.);
#7015=ORIENTED_EDGE('',*,*,#5267,.F.);
#7016=ORIENTED_EDGE('',*,*,#5228,.F.);
#7017=ORIENTED_EDGE('',*,*,#5266,.T.);
#7018=ORIENTED_EDGE('',*,*,#5268,.F.);
#7019=ORIENTED_EDGE('',*,*,#5269,.T.);
#7020=ORIENTED_EDGE('',*,*,#5270,.F.);
#7021=ORIENTED_EDGE('',*,*,#5271,.T.);
#7022=ORIENTED_EDGE('',*,*,#5272,.T.);
#7023=ORIENTED_EDGE('',*,*,#5237,.F.);
#7024=ORIENTED_EDGE('',*,*,#5267,.T.);
#7025=ORIENTED_EDGE('',*,*,#5211,.T.);
#7026=ORIENTED_EDGE('',*,*,#5270,.T.);
#7027=ORIENTED_EDGE('',*,*,#5273,.T.);
#7028=ORIENTED_EDGE('',*,*,#5238,.F.);
#7029=ORIENTED_EDGE('',*,*,#5274,.T.);
#7030=ORIENTED_EDGE('',*,*,#5259,.T.);
#7031=ORIENTED_EDGE('',*,*,#5222,.T.);
#7032=ORIENTED_EDGE('',*,*,#5263,.F.);
#7033=ORIENTED_EDGE('',*,*,#5261,.T.);
#7034=ORIENTED_EDGE('',*,*,#5254,.T.);
#7035=ORIENTED_EDGE('',*,*,#5235,.T.);
#7036=ORIENTED_EDGE('',*,*,#5272,.F.);
#7037=ORIENTED_EDGE('',*,*,#5275,.T.);
#7038=ORIENTED_EDGE('',*,*,#5250,.T.);
#7039=ORIENTED_EDGE('',*,*,#5255,.T.);
#7040=ORIENTED_EDGE('',*,*,#5275,.F.);
#7041=ORIENTED_EDGE('',*,*,#5271,.F.);
#7042=ORIENTED_EDGE('',*,*,#5274,.F.);
#7043=ORIENTED_EDGE('',*,*,#5241,.F.);
#7044=ORIENTED_EDGE('',*,*,#5244,.T.);
#7045=ORIENTED_EDGE('',*,*,#5247,.T.);
#7046=ORIENTED_EDGE('',*,*,#5248,.T.);
#7047=ORIENTED_EDGE('',*,*,#5245,.T.);
#7048=ORIENTED_EDGE('',*,*,#5242,.F.);
#7049=ORIENTED_EDGE('',*,*,#5239,.F.);
#7050=ORIENTED_EDGE('',*,*,#5273,.F.);
#7051=ORIENTED_EDGE('',*,*,#5269,.F.);
#7052=ORIENTED_EDGE('',*,*,#5276,.F.);
#7053=ORIENTED_EDGE('',*,*,#5251,.T.);
#7054=ORIENTED_EDGE('',*,*,#5276,.T.);
#7055=ORIENTED_EDGE('',*,*,#5268,.T.);
#7056=ORIENTED_EDGE('',*,*,#5210,.F.);
#7057=ORIENTED_EDGE('',*,*,#5252,.F.);
#8855=CYLINDRICAL_SURFACE('',#10014,6.34999999871023);
#8856=CYLINDRICAL_SURFACE('',#10017,6.34999999871025);
#8857=CYLINDRICAL_SURFACE('',#10020,6.34999999999997);
#8858=CYLINDRICAL_SURFACE('',#10023,6.98053323984749);
#8859=CYLINDRICAL_SURFACE('',#10026,6.35);
#8860=CYLINDRICAL_SURFACE('',#10029,6.34999999999999);
#8861=CYLINDRICAL_SURFACE('',#10032,6.35);
#8862=CYLINDRICAL_SURFACE('',#10035,6.35);
#8863=CYLINDRICAL_SURFACE('',#10058,4.);
#8864=CYLINDRICAL_SURFACE('',#10062,4.);
#8865=CYLINDRICAL_SURFACE('',#10064,4.);
#8866=CYLINDRICAL_SURFACE('',#10068,1.);
#8867=CYLINDRICAL_SURFACE('',#10070,1.);
#8868=CYLINDRICAL_SURFACE('',#10072,1.);
#9139=ADVANCED_FACE('',(#1000),#8855,.F.);
#9140=ADVANCED_FACE('',(#1001),#8856,.F.);
#9141=ADVANCED_FACE('',(#1002),#8857,.F.);
#9142=ADVANCED_FACE('',(#1003),#8858,.F.);
#9143=ADVANCED_FACE('',(#1004),#8859,.F.);
#9144=ADVANCED_FACE('',(#1005),#8860,.F.);
#9145=ADVANCED_FACE('',(#1006),#8861,.F.);
#9146=ADVANCED_FACE('',(#1007),#8862,.F.);
#9147=ADVANCED_FACE('',(#1008),#614,.T.);
#9148=ADVANCED_FACE('',(#1009),#615,.T.);
#9149=ADVANCED_FACE('',(#1010),#616,.T.);
#9150=ADVANCED_FACE('',(#1011),#617,.T.);
#9151=ADVANCED_FACE('',(#1012),#618,.T.);
#9152=ADVANCED_FACE('',(#1013),#619,.T.);
#9153=ADVANCED_FACE('',(#1014),#620,.T.);
#9154=ADVANCED_FACE('',(#1015),#621,.T.);
#9155=ADVANCED_FACE('',(#1016),#622,.T.);
#9156=ADVANCED_FACE('',(#1017),#623,.F.);
#9157=ADVANCED_FACE('',(#1018),#624,.T.);
#9158=ADVANCED_FACE('',(#1019),#625,.T.);
#9159=ADVANCED_FACE('',(#1020),#8863,.T.);
#9160=ADVANCED_FACE('',(#1021),#626,.T.);
#9161=ADVANCED_FACE('',(#1022),#8864,.T.);
#9162=ADVANCED_FACE('',(#1023,#417,#418,#419,#420),#627,.T.);
#9163=ADVANCED_FACE('',(#1024),#8865,.T.);
#9164=ADVANCED_FACE('',(#1025,#421,#422,#423,#424),#628,.T.);
#9165=ADVANCED_FACE('',(#1026),#629,.T.);
#9166=ADVANCED_FACE('',(#1027,#425,#426,#427,#428),#630,.F.);
#9167=ADVANCED_FACE('',(#1028),#8866,.F.);
#9168=ADVANCED_FACE('',(#1029,#429,#430,#431,#432),#631,.F.);
#9169=ADVANCED_FACE('',(#1030),#8867,.F.);
#9170=ADVANCED_FACE('',(#1031),#632,.F.);
#9171=ADVANCED_FACE('',(#1032),#8868,.F.);
#9172=ADVANCED_FACE('',(#1033),#633,.F.);
#9173=ADVANCED_FACE('',(#1034),#634,.F.);
#9174=ADVANCED_FACE('',(#1035),#635,.F.);
#9175=ADVANCED_FACE('',(#1036),#636,.F.);
#9176=ADVANCED_FACE('',(#1037),#637,.T.);
#9558=CLOSED_SHELL('',(#9139,#9140,#9141,#9142,#9143,#9144,#9145,#9146,
#9147,#9148,#9149,#9150,#9151,#9152,#9153,#9154,#9155,#9156,#9157,#9158,
#9159,#9160,#9161,#9162,#9163,#9164,#9165,#9166,#9167,#9168,#9169,#9170,
#9171,#9172,#9173,#9174,#9175,#9176));
#10013=AXIS2_PLACEMENT_3D('',#14538,#11648,#11649);
#10014=AXIS2_PLACEMENT_3D('',#14539,#11650,#11651);
#10015=AXIS2_PLACEMENT_3D('',#14541,#11652,#11653);
#10016=AXIS2_PLACEMENT_3D('',#14544,#11655,#11656);
#10017=AXIS2_PLACEMENT_3D('',#14545,#11657,#11658);
#10018=AXIS2_PLACEMENT_3D('',#14547,#11659,#11660);
#10019=AXIS2_PLACEMENT_3D('',#14550,#11662,#11663);
#10020=AXIS2_PLACEMENT_3D('',#14551,#11664,#11665);
#10021=AXIS2_PLACEMENT_3D('',#14553,#11666,#11667);
#10022=AXIS2_PLACEMENT_3D('',#14556,#11669,#11670);
#10023=AXIS2_PLACEMENT_3D('',#14557,#11671,#11672);
#10024=AXIS2_PLACEMENT_3D('',#14559,#11673,#11674);
#10025=AXIS2_PLACEMENT_3D('',#14562,#11676,#11677);
#10026=AXIS2_PLACEMENT_3D('',#14563,#11678,#11679);
#10027=AXIS2_PLACEMENT_3D('',#14565,#11680,#11681);
#10028=AXIS2_PLACEMENT_3D('',#14568,#11683,#11684);
#10029=AXIS2_PLACEMENT_3D('',#14569,#11685,#11686);
#10030=AXIS2_PLACEMENT_3D('',#14571,#11687,#11688);
#10031=AXIS2_PLACEMENT_3D('',#14574,#11690,#11691);
#10032=AXIS2_PLACEMENT_3D('',#14575,#11692,#11693);
#10033=AXIS2_PLACEMENT_3D('',#14577,#11694,#11695);
#10034=AXIS2_PLACEMENT_3D('',#14580,#11697,#11698);
#10035=AXIS2_PLACEMENT_3D('',#14581,#11699,#11700);
#10036=AXIS2_PLACEMENT_3D('',#14583,#11701,#11702);
#10037=AXIS2_PLACEMENT_3D('',#14586,#11704,#11705);
#10038=AXIS2_PLACEMENT_3D('',#14587,#11706,#11707);
#10039=AXIS2_PLACEMENT_3D('',#14596,#11712,#11713);
#10040=AXIS2_PLACEMENT_3D('',#14601,#11715,#11716);
#10041=AXIS2_PLACEMENT_3D('',#14604,#11718,#11719);
#10042=AXIS2_PLACEMENT_3D('',#14605,#11720,#11721);
#10043=AXIS2_PLACEMENT_3D('',#14611,#11725,#11726);
#10044=AXIS2_PLACEMENT_3D('',#14616,#11728,#11729);
#10045=AXIS2_PLACEMENT_3D('',#14619,#11731,#11732);
#10046=AXIS2_PLACEMENT_3D('',#14620,#11733,#11734);
#10047=AXIS2_PLACEMENT_3D('',#14626,#11738,#11739);
#10048=AXIS2_PLACEMENT_3D('',#14631,#11741,#11742);
#10049=AXIS2_PLACEMENT_3D('',#14634,#11744,#11745);
#10050=AXIS2_PLACEMENT_3D('',#14635,#11746,#11747);
#10051=AXIS2_PLACEMENT_3D('',#14638,#11750,#11751);
#10052=AXIS2_PLACEMENT_3D('',#14639,#11752,#11753);
#10053=AXIS2_PLACEMENT_3D('',#14640,#11754,#11755);
#10054=AXIS2_PLACEMENT_3D('',#14641,#11756,#11757);
#10055=AXIS2_PLACEMENT_3D('',#14647,#11761,#11762);
#10056=AXIS2_PLACEMENT_3D('',#14656,#11767,#11768);
#10057=AXIS2_PLACEMENT_3D('',#14662,#11772,#11773);
#10058=AXIS2_PLACEMENT_3D('',#14668,#11777,#11778);
#10059=AXIS2_PLACEMENT_3D('',#14670,#11779,#11780);
#10060=AXIS2_PLACEMENT_3D('',#14673,#11782,#11783);
#10061=AXIS2_PLACEMENT_3D('',#14674,#11784,#11785);
#10062=AXIS2_PLACEMENT_3D('',#14682,#11791,#11792);
#10063=AXIS2_PLACEMENT_3D('',#14684,#11794,#11795);
#10064=AXIS2_PLACEMENT_3D('',#14686,#11797,#11798);
#10065=AXIS2_PLACEMENT_3D('',#14688,#11800,#11801);
#10066=AXIS2_PLACEMENT_3D('',#14692,#11804,#11805);
#10067=AXIS2_PLACEMENT_3D('',#14696,#11808,#11809);
#10068=AXIS2_PLACEMENT_3D('',#14699,#11812,#11813);
#10069=AXIS2_PLACEMENT_3D('',#14701,#11815,#11816);
#10070=AXIS2_PLACEMENT_3D('',#14703,#11818,#11819);
#10071=AXIS2_PLACEMENT_3D('',#14705,#11821,#11822);
#10072=AXIS2_PLACEMENT_3D('',#14715,#11828,#11829);
#10073=AXIS2_PLACEMENT_3D('',#14716,#11830,#11831);
#10074=AXIS2_PLACEMENT_3D('',#14717,#11832,#11833);
#10075=AXIS2_PLACEMENT_3D('',#14718,#11834,#11835);
#10076=AXIS2_PLACEMENT_3D('',#14719,#11836,#11837);
#10077=AXIS2_PLACEMENT_3D('',#14721,#11839,#11840);
#10078=AXIS2_PLACEMENT_3D('',#14722,#11841,#11842);
#10079=AXIS2_PLACEMENT_3D('',#14724,#11844,#11845);
#11648=DIRECTION('axis',(0.,0.,1.));
#11649=DIRECTION('refdir',(1.,0.,0.));
#11650=DIRECTION('center_axis',(-1.,0.,0.));
#11651=DIRECTION('ref_axis',(0.,0.,1.));
#11652=DIRECTION('center_axis',(-1.,0.,0.));
#11653=DIRECTION('ref_axis',(0.,0.,1.));
#11654=DIRECTION('',(-1.,0.,0.));
#11655=DIRECTION('center_axis',(-1.,0.,0.));
#11656=DIRECTION('ref_axis',(0.,0.,1.));
#11657=DIRECTION('center_axis',(-1.,0.,0.));
#11658=DIRECTION('ref_axis',(0.,0.,1.));
#11659=DIRECTION('center_axis',(-1.,0.,0.));
#11660=DIRECTION('ref_axis',(0.,0.,1.));
#11661=DIRECTION('',(-1.,0.,0.));
#11662=DIRECTION('center_axis',(-1.,0.,0.));
#11663=DIRECTION('ref_axis',(0.,0.,1.));
#11664=DIRECTION('center_axis',(-1.,0.,0.));
#11665=DIRECTION('ref_axis',(0.,0.,1.));
#11666=DIRECTION('center_axis',(-1.,0.,0.));
#11667=DIRECTION('ref_axis',(0.,0.,1.));
#11668=DIRECTION('',(-1.,0.,0.));
#11669=DIRECTION('center_axis',(-1.,0.,0.));
#11670=DIRECTION('ref_axis',(0.,0.,1.));
#11671=DIRECTION('center_axis',(-1.,0.,0.));
#11672=DIRECTION('ref_axis',(0.,0.,1.));
#11673=DIRECTION('center_axis',(-1.,0.,0.));
#11674=DIRECTION('ref_axis',(0.,0.,1.));
#11675=DIRECTION('',(-1.,0.,0.));
#11676=DIRECTION('center_axis',(-1.,0.,0.));
#11677=DIRECTION('ref_axis',(0.,0.,1.));
#11678=DIRECTION('center_axis',(1.22464679914735E-16,-1.,0.));
#11679=DIRECTION('ref_axis',(1.,1.22464679914735E-16,0.));
#11680=DIRECTION('center_axis',(1.22464679914735E-16,-1.,0.));
#11681=DIRECTION('ref_axis',(1.,1.22464679914735E-16,0.));
#11682=DIRECTION('',(1.22464679914735E-16,-1.,0.));
#11683=DIRECTION('center_axis',(1.22464679914735E-16,-1.,0.));
#11684=DIRECTION('ref_axis',(1.,1.22464679914735E-16,0.));
#11685=DIRECTION('center_axis',(1.22464679914735E-16,-1.,0.));
#11686=DIRECTION('ref_axis',(1.,1.22464679914735E-16,0.));
#11687=DIRECTION('center_axis',(1.22464679914735E-16,-1.,0.));
#11688=DIRECTION('ref_axis',(1.,1.22464679914735E-16,0.));
#11689=DIRECTION('',(1.22464679914735E-16,-1.,0.));
#11690=DIRECTION('center_axis',(1.22464679914735E-16,-1.,0.));
#11691=DIRECTION('ref_axis',(-1.,-1.22464679914735E-16,0.));
#11692=DIRECTION('center_axis',(1.22464679914735E-16,-1.,0.));
#11693=DIRECTION('ref_axis',(1.,1.22464679914735E-16,0.));
#11694=DIRECTION('center_axis',(1.22464679914735E-16,-1.,0.));
#11695=DIRECTION('ref_axis',(1.,1.22464679914735E-16,0.));
#11696=DIRECTION('',(1.22464679914735E-16,-1.,0.));
#11697=DIRECTION('center_axis',(1.22464679914735E-16,-1.,0.));
#11698=DIRECTION('ref_axis',(1.,1.22464679914735E-16,0.));
#11699=DIRECTION('center_axis',(1.22464679914735E-16,-1.,0.));
#11700=DIRECTION('ref_axis',(1.,1.22464679914735E-16,0.));
#11701=DIRECTION('center_axis',(1.22464679914735E-16,-1.,0.));
#11702=DIRECTION('ref_axis',(1.,1.22464679914735E-16,0.));
#11703=DIRECTION('',(1.22464679914735E-16,-1.,0.));
#11704=DIRECTION('center_axis',(1.22464679914735E-16,-1.,0.));
#11705=DIRECTION('ref_axis',(1.,1.22464679914735E-16,0.));
#11706=DIRECTION('center_axis',(0.,0.,-1.));
#11707=DIRECTION('ref_axis',(-1.,0.,0.));
#11708=DIRECTION('',(1.,0.,0.));
#11709=DIRECTION('',(0.,-1.,0.));
#11710=DIRECTION('',(1.,0.,0.));
#11711=DIRECTION('',(0.,1.,0.));
#11712=DIRECTION('center_axis',(0.,0.,1.));
#11713=DIRECTION('ref_axis',(1.,0.,0.));
#11714=DIRECTION('',(0.,-1.,0.));
#11715=DIRECTION('center_axis',(0.,0.,-1.));
#11716=DIRECTION('ref_axis',(1.,0.,0.));
#11717=DIRECTION('',(1.,0.,0.));
#11718=DIRECTION('center_axis',(0.,0.,-1.));
#11719=DIRECTION('ref_axis',(1.,0.,0.));
#11720=DIRECTION('center_axis',(0.,0.,1.));
#11721=DIRECTION('ref_axis',(1.,0.,0.));
#11722=DIRECTION('',(-1.,-1.22464679914735E-16,0.));
#11723=DIRECTION('',(-1.,-1.22464679914735E-16,0.));
#11724=DIRECTION('',(1.22464679914735E-16,-1.,0.));
#11725=DIRECTION('center_axis',(0.,0.,-1.));
#11726=DIRECTION('ref_axis',(-1.,0.,0.));
#11727=DIRECTION('',(-1.,0.,0.));
#11728=DIRECTION('center_axis',(0.,0.,-1.));
#11729=DIRECTION('ref_axis',(1.,0.,0.));
#11730=DIRECTION('',(0.,1.,0.));
#11731=DIRECTION('center_axis',(0.,0.,-1.));
#11732=DIRECTION('ref_axis',(1.,0.,0.));
#11733=DIRECTION('center_axis',(0.,0.,-1.));
#11734=DIRECTION('ref_axis',(-1.,0.,0.));
#11735=DIRECTION('',(0.,1.,0.));
#11736=DIRECTION('',(0.,1.,0.));
#11737=DIRECTION('',(1.,0.,0.));
#11738=DIRECTION('center_axis',(0.,0.,1.));
#11739=DIRECTION('ref_axis',(1.,0.,0.));
#11740=DIRECTION('',(-1.,0.,0.));
#11741=DIRECTION('center_axis',(0.,0.,-1.));
#11742=DIRECTION('ref_axis',(1.,0.,0.));
#11743=DIRECTION('',(0.,-1.,0.));
#11744=DIRECTION('center_axis',(0.,0.,-1.));
#11745=DIRECTION('ref_axis',(1.,0.,0.));
#11746=DIRECTION('center_axis',(0.,0.,1.));
#11747=DIRECTION('ref_axis',(1.,0.,0.));
#11748=DIRECTION('',(0.,1.,0.));
#11749=DIRECTION('',(0.,1.,0.));
#11750=DIRECTION('center_axis',(0.,0.,-1.));
#11751=DIRECTION('ref_axis',(-1.,0.,0.));
#11752=DIRECTION('center_axis',(0.,0.,-1.));
#11753=DIRECTION('ref_axis',(1.,0.,0.));
#11754=DIRECTION('center_axis',(0.,0.,-1.));
#11755=DIRECTION('ref_axis',(1.,0.,0.));
#11756=DIRECTION('center_axis',(0.,0.,1.));
#11757=DIRECTION('ref_axis',(1.,0.,0.));
#11758=DIRECTION('',(0.,-1.,0.));
#11759=DIRECTION('',(1.,0.,0.));
#11760=DIRECTION('',(1.,0.,0.));
#11761=DIRECTION('center_axis',(1.,-3.65204942310907E-16,0.));
#11762=DIRECTION('ref_axis',(3.65204942310907E-16,1.,0.));
#11763=DIRECTION('',(0.,0.,-1.));
#11764=DIRECTION('',(-1.68975972140531E-16,-0.462688076101332,0.886521147087675));
#11765=DIRECTION('',(0.,0.,-1.));
#11766=DIRECTION('',(1.71139076064604E-16,0.468611062549393,0.883404591371547));
#11767=DIRECTION('center_axis',(0.,-1.,0.));
#11768=DIRECTION('ref_axis',(0.,0.,-1.));
#11769=DIRECTION('',(1.,0.,0.));
#11770=DIRECTION('',(0.,0.,-1.));
#11771=DIRECTION('',(1.,0.,0.));
#11772=DIRECTION('center_axis',(1.,-3.65204942310907E-16,0.));
#11773=DIRECTION('ref_axis',(3.65204942310907E-16,1.,0.));
#11774=DIRECTION('',(0.,-0.462688076101332,0.886521147087675));
#11775=DIRECTION('',(0.,0.,-1.));
#11776=DIRECTION('',(0.,0.468611062549393,0.883404591371547));
#11777=DIRECTION('center_axis',(0.,0.,-1.));
#11778=DIRECTION('ref_axis',(0.707106781186548,0.707106781186547,0.));
#11779=DIRECTION('center_axis',(-9.04452389970748E-15,-0.886521147087677,
-0.462688076101329));
#11780=DIRECTION('ref_axis',(8.69090002824443E-14,0.462688076101329,-0.886521147087677));
#11781=DIRECTION('',(0.,0.,-1.));
#11782=DIRECTION('center_axis',(-1.79450933059916E-14,-0.88340459137155,
0.468611062549386));
#11783=DIRECTION('ref_axis',(1.21092278199327E-14,-0.468611062549386,-0.88340459137155));
#11784=DIRECTION('center_axis',(0.,1.,0.));
#11785=DIRECTION('ref_axis',(0.,0.,1.));
#11786=DIRECTION('',(1.,0.,0.));
#11787=DIRECTION('',(0.,0.,-1.));
#11788=DIRECTION('',(0.,0.,-1.));
#11789=DIRECTION('',(0.,0.,1.));
#11790=DIRECTION('',(-1.,0.,0.));
#11791=DIRECTION('center_axis',(0.,0.,-1.));
#11792=DIRECTION('ref_axis',(-1.,0.,0.));
#11793=DIRECTION('',(0.,0.,-1.));
#11794=DIRECTION('center_axis',(-1.,0.,0.));
#11795=DIRECTION('ref_axis',(0.,0.,1.));
#11796=DIRECTION('',(0.,0.,-1.));
#11797=DIRECTION('center_axis',(0.,0.,-1.));
#11798=DIRECTION('ref_axis',(-1.,0.,0.));
#11799=DIRECTION('',(0.,0.,-1.));
#11800=DIRECTION('center_axis',(1.22464679914735E-16,-1.,0.));
#11801=DIRECTION('ref_axis',(1.,1.22464679914735E-16,0.));
#11802=DIRECTION('',(-1.,-1.22464679914735E-16,0.));
#11803=DIRECTION('',(0.,0.,-1.));
#11804=DIRECTION('center_axis',(1.,1.22464679914735E-16,0.));
#11805=DIRECTION('ref_axis',(-1.22464679914735E-16,1.,0.));
#11806=DIRECTION('',(1.22464679914735E-16,-1.,0.));
#11807=DIRECTION('',(0.,0.,-1.));
#11808=DIRECTION('center_axis',(1.22464679914735E-16,-1.,0.));
#11809=DIRECTION('ref_axis',(1.,1.22464679914735E-16,0.));
#11810=DIRECTION('',(-1.,-1.22464679914735E-16,0.));
#11811=DIRECTION('',(0.,0.,-1.));
#11812=DIRECTION('center_axis',(0.,0.,-1.));
#11813=DIRECTION('ref_axis',(-1.,0.,0.));
#11814=DIRECTION('',(0.,0.,-1.));
#11815=DIRECTION('center_axis',(-1.,0.,0.));
#11816=DIRECTION('ref_axis',(0.,0.,1.));
#11817=DIRECTION('',(0.,0.,-1.));
#11818=DIRECTION('center_axis',(0.,0.,-1.));
#11819=DIRECTION('ref_axis',(-1.,0.,0.));
#11820=DIRECTION('',(0.,0.,-1.));
#11821=DIRECTION('center_axis',(0.,1.,0.));
#11822=DIRECTION('ref_axis',(0.,0.,1.));
#11823=DIRECTION('',(0.,0.,-1.));
#11824=DIRECTION('',(1.,0.,0.));
#11825=DIRECTION('',(0.,0.,-1.));
#11826=DIRECTION('',(-1.,0.,0.));
#11827=DIRECTION('',(0.,0.,1.));
#11828=DIRECTION('center_axis',(0.,0.,-1.));
#11829=DIRECTION('ref_axis',(-1.,0.,0.));
#11830=DIRECTION('center_axis',(-2.77796091205298E-14,-0.886521147087676,
-0.462688076101331));
#11831=DIRECTION('ref_axis',(6.62185632336808E-14,0.462688076101331,-0.886521147087676));
#11832=DIRECTION('center_axis',(1.88700981155792E-14,-0.883404591371546,
0.468611062549393));
#11833=DIRECTION('ref_axis',(3.43055792298147E-13,-0.468611062549393,-0.883404591371546));
#11834=DIRECTION('center_axis',(0.,0.,1.));
#11835=DIRECTION('ref_axis',(1.,0.,0.));
#11836=DIRECTION('center_axis',(-1.,0.,0.));
#11837=DIRECTION('ref_axis',(0.,0.,1.));
#11838=DIRECTION('',(0.,0.468611062549393,0.883404591371547));
#11839=DIRECTION('center_axis',(0.,0.883404591371547,-0.468611062549393));
#11840=DIRECTION('ref_axis',(0.,0.468611062549393,0.883404591371547));
#11841=DIRECTION('center_axis',(0.,0.886521147087676,0.462688076101332));
#11842=DIRECTION('ref_axis',(0.,-0.462688076101332,0.886521147087676));
#11843=DIRECTION('',(0.,-0.462688076101332,0.886521147087675));
#11844=DIRECTION('center_axis',(1.,0.,0.));
#11845=DIRECTION('ref_axis',(0.,0.,-1.));
#14538=CARTESIAN_POINT('',(0.,0.,0.));
#14539=CARTESIAN_POINT('Origin',(-81.58,34.5,63.9999999999928));
#14540=CARTESIAN_POINT('',(-82.,34.5,57.6500000012826));
#14541=CARTESIAN_POINT('Origin',(-82.,34.5,63.9999999999928));
#14542=CARTESIAN_POINT('',(-85.,34.5,57.6500000012826));
#14543=CARTESIAN_POINT('',(-81.58,34.5,57.6500000012826));
#14544=CARTESIAN_POINT('Origin',(-85.,34.5,63.9999999999928));
#14545=CARTESIAN_POINT('Origin',(-81.58,34.5,138.999999999993));
#14546=CARTESIAN_POINT('',(-82.,34.5,132.650000001283));
#14547=CARTESIAN_POINT('Origin',(-82.,34.5,138.999999999993));
#14548=CARTESIAN_POINT('',(-85.,34.5,132.650000001283));
#14549=CARTESIAN_POINT('',(-81.58,34.5,132.650000001283));
#14550=CARTESIAN_POINT('Origin',(-85.,34.5,138.999999999993));
#14551=CARTESIAN_POINT('Origin',(-81.58,37.8359855953527,608.));
#14552=CARTESIAN_POINT('',(-82.,37.8359855953527,601.65));
#14553=CARTESIAN_POINT('Origin',(-82.,37.8359855953527,608.));
#14554=CARTESIAN_POINT('',(-85.,37.8359855953527,601.65));
#14555=CARTESIAN_POINT('',(-81.58,37.8359855953527,601.65));
#14556=CARTESIAN_POINT('Origin',(-85.,37.8359855953527,608.));
#14557=CARTESIAN_POINT('Origin',(-81.58,35.9826602646012,683.));
#14558=CARTESIAN_POINT('',(-82.,35.9826602646012,676.019466760152));
#14559=CARTESIAN_POINT('Origin',(-82.,35.9826602646012,683.));
#14560=CARTESIAN_POINT('',(-85.,35.9826602646012,676.019466760152));
#14561=CARTESIAN_POINT('',(-81.58,35.9826602646012,676.019466760152));
#14562=CARTESIAN_POINT('Origin',(-85.,35.9826602646012,683.));
#14563=CARTESIAN_POINT('Origin',(-42.5,1.49999999999999,32.0000000000144));
#14564=CARTESIAN_POINT('',(-48.85,-6.10622663543836E-15,32.0000000000144));
#14565=CARTESIAN_POINT('Origin',(-42.5,-5.20417042793042E-15,32.0000000000144));
#14566=CARTESIAN_POINT('',(-48.85,-3.00000000000001,32.0000000000144));
#14567=CARTESIAN_POINT('',(-48.85,1.49999999999999,32.0000000000144));
#14568=CARTESIAN_POINT('Origin',(-42.5,-3.00000000000001,32.0000000000144));
#14569=CARTESIAN_POINT('Origin',(-42.5000000000001,1.49999999999999,713.999999999986));
#14570=CARTESIAN_POINT('',(-48.8500000000001,-6.10622663543836E-15,713.999999999986));
#14571=CARTESIAN_POINT('Origin',(-42.5000000000001,-5.20417042793042E-15,
713.999999999986));
#14572=CARTESIAN_POINT('',(-48.8500000000001,-3.00000000000001,713.999999999986));
#14573=CARTESIAN_POINT('',(-48.8500000000001,1.49999999999999,713.999999999986));
#14574=CARTESIAN_POINT('Origin',(-42.5000000000001,-3.00000000000001,713.999999999986));
#14575=CARTESIAN_POINT('Origin',(-42.2900000000001,1.49999999999999,529.5));
#14576=CARTESIAN_POINT('',(-48.6400000000001,-6.10622663543836E-15,529.5));
#14577=CARTESIAN_POINT('Origin',(-42.2900000000001,-5.20417042793042E-15,
529.5));
#14578=CARTESIAN_POINT('',(-48.6400000000001,-3.00000000000001,529.5));
#14579=CARTESIAN_POINT('',(-48.6400000000001,1.49999999999999,529.5));
#14580=CARTESIAN_POINT('Origin',(-42.2900000000001,-3.00000000000001,529.5));
#14581=CARTESIAN_POINT('Origin',(-42.5,1.49999999999999,175.500000000014));
#14582=CARTESIAN_POINT('',(-48.85,-6.10622663543836E-15,175.500000000014));
#14583=CARTESIAN_POINT('Origin',(-42.5,-5.20417042793042E-15,175.500000000014));
#14584=CARTESIAN_POINT('',(-48.85,-3.00000000000001,175.500000000014));
#14585=CARTESIAN_POINT('',(-48.85,1.49999999999999,175.500000000014));
#14586=CARTESIAN_POINT('Origin',(-42.5,-3.00000000000001,175.500000000014));
#14587=CARTESIAN_POINT('Origin',(-85.,68.,0.));
#14588=CARTESIAN_POINT('',(-81.,72.,0.));
#14589=CARTESIAN_POINT('',(-33.5,72.,0.));
#14590=CARTESIAN_POINT('',(-82.,72.,0.));
#14591=CARTESIAN_POINT('',(-33.5,69.,0.));
#14592=CARTESIAN_POINT('',(-33.5,68.,0.));
#14593=CARTESIAN_POINT('',(-81.,69.,0.));
#14594=CARTESIAN_POINT('',(-82.,69.,0.));
#14595=CARTESIAN_POINT('',(-81.,69.,0.));
#14596=CARTESIAN_POINT('Origin',(-81.,-9.91963907309357E-15,746.));
#14597=CARTESIAN_POINT('',(-81.,-9.91963907309357E-15,746.));
#14598=CARTESIAN_POINT('',(-81.,-3.00000000000001,746.));
#14599=CARTESIAN_POINT('',(-81.,-9.91963907309357E-15,746.));
#14600=CARTESIAN_POINT('',(-82.,0.99999999999999,746.));
#14601=CARTESIAN_POINT('Origin',(-81.,0.99999999999999,746.));
#14602=CARTESIAN_POINT('',(-85.,0.99999999999999,746.));
#14603=CARTESIAN_POINT('',(-85.,0.99999999999999,746.));
#14604=CARTESIAN_POINT('Origin',(-81.,0.99999999999999,746.));
#14605=CARTESIAN_POINT('Origin',(-85.,0.99999999999999,746.));
#14606=CARTESIAN_POINT('',(0.,0.,746.));
#14607=CARTESIAN_POINT('',(0.,0.,746.));
#14608=CARTESIAN_POINT('',(3.67394039744206E-16,-3.,746.));
#14609=CARTESIAN_POINT('',(3.67394039744206E-16,-3.,746.));
#14610=CARTESIAN_POINT('',(0.,0.,746.));
#14611=CARTESIAN_POINT('Origin',(-82.,0.99999999999999,0.));
#14612=CARTESIAN_POINT('',(-82.,0.99999999999999,0.));
#14613=CARTESIAN_POINT('',(-85.,0.99999999999999,0.));
#14614=CARTESIAN_POINT('',(-82.,0.99999999999999,0.));
#14615=CARTESIAN_POINT('',(-81.,-9.91963907309357E-15,0.));
#14616=CARTESIAN_POINT('Origin',(-81.,0.99999999999999,0.));
#14617=CARTESIAN_POINT('',(-81.,-3.00000000000001,0.));
#14618=CARTESIAN_POINT('',(-81.,-3.00000000000001,0.));
#14619=CARTESIAN_POINT('Origin',(-81.,0.99999999999999,0.));
#14620=CARTESIAN_POINT('Origin',(-81.,-3.00000000000001,0.));
#14621=CARTESIAN_POINT('',(-82.,68.,0.));
#14622=CARTESIAN_POINT('',(-82.,-1.00421037530083E-14,0.));
#14623=CARTESIAN_POINT('',(-85.,68.,0.));
#14624=CARTESIAN_POINT('',(-85.,-1.00421037530083E-14,0.));
#14625=CARTESIAN_POINT('',(-85.,68.,0.));
#14626=CARTESIAN_POINT('Origin',(-82.,68.,746.));
#14627=CARTESIAN_POINT('',(-82.,68.,746.));
#14628=CARTESIAN_POINT('',(-85.,68.,746.));
#14629=CARTESIAN_POINT('',(-82.,68.,746.));
#14630=CARTESIAN_POINT('',(-81.,69.,746.));
#14631=CARTESIAN_POINT('Origin',(-81.,68.,746.));
#14632=CARTESIAN_POINT('',(-81.,72.,746.));
#14633=CARTESIAN_POINT('',(-81.,72.,746.));
#14634=CARTESIAN_POINT('Origin',(-81.,68.,746.));
#14635=CARTESIAN_POINT('Origin',(-81.,72.,746.));
#14636=CARTESIAN_POINT('',(-82.,-1.00421037530083E-14,746.));
#14637=CARTESIAN_POINT('',(-85.,-1.00421037530083E-14,746.));
#14638=CARTESIAN_POINT('Origin',(-81.,69.,0.));
#14639=CARTESIAN_POINT('Origin',(-81.,68.,0.));
#14640=CARTESIAN_POINT('Origin',(-81.,68.,0.));
#14641=CARTESIAN_POINT('Origin',(-29.,68.,746.));
#14642=CARTESIAN_POINT('',(-33.5,72.,746.));
#14643=CARTESIAN_POINT('',(-33.5,69.,746.));
#14644=CARTESIAN_POINT('',(-33.5,50.,746.));
#14645=CARTESIAN_POINT('',(-82.,72.,746.));
#14646=CARTESIAN_POINT('',(-82.,69.,746.));
#14647=CARTESIAN_POINT('Origin',(-32.,69.,746.));
#14648=CARTESIAN_POINT('',(-32.,68.,565.447580013871));
#14649=CARTESIAN_POINT('',(-32.,68.,139.329431198143));
#14650=CARTESIAN_POINT('',(-32.,68.,746.));
#14651=CARTESIAN_POINT('',(-32.,50.,173.817851090086));
#14652=CARTESIAN_POINT('',(-32.0000000000001,-180.631730474111,615.713626701011));
#14653=CARTESIAN_POINT('',(-32.,50.,531.514786028642));
#14654=CARTESIAN_POINT('',(-32.,50.,746.));
#14655=CARTESIAN_POINT('',(-32.,142.963452937836,706.765324733926));
#14656=CARTESIAN_POINT('Origin',(-29.,50.,746.));
#14657=CARTESIAN_POINT('',(-29.,50.,173.817851090086));
#14658=CARTESIAN_POINT('',(-33.5,50.,173.817851090086));
#14659=CARTESIAN_POINT('',(-29.,50.,531.514786028642));
#14660=CARTESIAN_POINT('',(-29.,50.,746.));
#14661=CARTESIAN_POINT('',(-33.5,50.,531.514786028642));
#14662=CARTESIAN_POINT('Origin',(-29.,69.,746.));
#14663=CARTESIAN_POINT('',(-29.,68.,139.329431198143));
#14664=CARTESIAN_POINT('',(-29.,50.,173.817851090086));
#14665=CARTESIAN_POINT('',(-29.,68.,565.447580013871));
#14666=CARTESIAN_POINT('',(-29.,68.,746.));
#14667=CARTESIAN_POINT('',(-29.,72.6655742581807,574.242911687517));
#14668=CARTESIAN_POINT('Origin',(-33.,68.,746.));
#14669=CARTESIAN_POINT('',(-33.,72.,131.665337888822));
#14670=CARTESIAN_POINT('Origin',(-33.0000000000006,67.9999999999993,139.329431198144));
#14671=CARTESIAN_POINT('',(-33.,72.,572.988200899477));
#14672=CARTESIAN_POINT('',(-33.,72.,746.));
#14673=CARTESIAN_POINT('Origin',(-32.9999999999998,68.0000000000002,565.447580013871));
#14674=CARTESIAN_POINT('Origin',(-82.,72.,746.));
#14675=CARTESIAN_POINT('',(-33.5,72.,131.665337888822));
#14676=CARTESIAN_POINT('',(-82.,72.,131.665337888822));
#14677=CARTESIAN_POINT('',(-33.5,72.,746.));
#14678=CARTESIAN_POINT('',(-81.,72.,746.));
#14679=CARTESIAN_POINT('',(-33.5,72.,572.988200899477));
#14680=CARTESIAN_POINT('',(-33.5,72.,746.));
#14681=CARTESIAN_POINT('',(-82.,72.,572.988200899477));
#14682=CARTESIAN_POINT('Origin',(-81.,68.,746.));
#14683=CARTESIAN_POINT('',(-85.,68.,746.));
#14684=CARTESIAN_POINT('Origin',(-85.,-1.00421037530083E-14,746.));
#14685=CARTESIAN_POINT('',(-85.,0.99999999999999,746.));
#14686=CARTESIAN_POINT('Origin',(-81.,0.99999999999999,746.));
#14687=CARTESIAN_POINT('',(-81.,-3.00000000000001,746.));
#14688=CARTESIAN_POINT('Origin',(3.67394039744206E-16,-3.,746.));
#14689=CARTESIAN_POINT('',(3.67394039744206E-16,-3.,0.));
#14690=CARTESIAN_POINT('',(3.67394039744206E-16,-3.,0.));
#14691=CARTESIAN_POINT('',(3.67394039744206E-16,-3.,746.));
#14692=CARTESIAN_POINT('Origin',(0.,0.,746.));
#14693=CARTESIAN_POINT('',(0.,0.,0.));
#14694=CARTESIAN_POINT('',(0.,0.,0.));
#14695=CARTESIAN_POINT('',(0.,0.,746.));
#14696=CARTESIAN_POINT('Origin',(0.,0.,746.));
#14697=CARTESIAN_POINT('',(0.,0.,0.));
#14698=CARTESIAN_POINT('',(-81.,-9.91963907309357E-15,746.));
#14699=CARTESIAN_POINT('Origin',(-81.,0.99999999999999,746.));
#14700=CARTESIAN_POINT('',(-82.,0.99999999999999,746.));
#14701=CARTESIAN_POINT('Origin',(-82.,-1.00421037530083E-14,746.));
#14702=CARTESIAN_POINT('',(-82.,68.,746.));
#14703=CARTESIAN_POINT('Origin',(-81.,68.,746.));
#14704=CARTESIAN_POINT('',(-81.,69.,746.));
#14705=CARTESIAN_POINT('Origin',(-82.,69.,746.));
#14706=CARTESIAN_POINT('',(-33.5,69.,137.413407870812));
#14707=CARTESIAN_POINT('',(-33.5,69.,746.));
#14708=CARTESIAN_POINT('',(-33.,69.,137.413407870813));
#14709=CARTESIAN_POINT('',(-82.,69.,137.413407870813));
#14710=CARTESIAN_POINT('',(-33.,69.,567.332735235272));
#14711=CARTESIAN_POINT('',(-33.,69.,746.));
#14712=CARTESIAN_POINT('',(-33.5,69.,567.332735235272));
#14713=CARTESIAN_POINT('',(-82.,69.,567.332735235272));
#14714=CARTESIAN_POINT('',(-33.5,69.,746.));
#14715=CARTESIAN_POINT('Origin',(-33.,68.,746.));
#14716=CARTESIAN_POINT('Origin',(-33.0000000000001,67.9999999999998,139.329431198143));
#14717=CARTESIAN_POINT('Origin',(-32.9999999999994,68.0000000000007,565.447580013872));
#14718=CARTESIAN_POINT('Origin',(-33.,68.,0.));
#14719=CARTESIAN_POINT('Origin',(-33.5,0.,0.));
#14720=CARTESIAN_POINT('',(-33.5,72.6655742581807,574.242911687517));
#14721=CARTESIAN_POINT('Origin',(-33.5,72.6655742581807,574.242911687517));
#14722=CARTESIAN_POINT('Origin',(-33.5,50.,173.817851090086));
#14723=CARTESIAN_POINT('',(-33.5,50.,173.817851090086));
#14724=CARTESIAN_POINT('Origin',(-33.5,0.,0.));
#17970=UNCERTAINTY_MEASURE_WITH_UNIT(LENGTH_MEASURE(0.01),#18007,
'DISTANCE_ACCURACY_VALUE',
'Maximum model space distance between geometric entities at asserted c
onnectivities');
#17986=UNCERTAINTY_MEASURE_WITH_UNIT(LENGTH_MEASURE(0.01),#18007,
'DISTANCE_ACCURACY_VALUE',
'Maximum model space distance between geometric entities at asserted c
onnectivities');
#17990=(
GEOMETRIC_REPRESENTATION_CONTEXT(3)
GLOBAL_UNCERTAINTY_ASSIGNED_CONTEXT((#17970))
GLOBAL_UNIT_ASSIGNED_CONTEXT((#18007,#18009,#18010))
REPRESENTATION_CONTEXT('','3D')
);
#18006=(
GEOMETRIC_REPRESENTATION_CONTEXT(3)
GLOBAL_UNCERTAINTY_ASSIGNED_CONTEXT((#17986))
GLOBAL_UNIT_ASSIGNED_CONTEXT((#18007,#18009,#18010))
REPRESENTATION_CONTEXT('','3D')
);
#18007=(
LENGTH_UNIT()
NAMED_UNIT(*)
SI_UNIT(.MILLI.,.METRE.)
);
#18009=(
NAMED_UNIT(*)
PLANE_ANGLE_UNIT()
SI_UNIT($,.RADIAN.)
);
#18010=(
NAMED_UNIT(*)
SI_UNIT($,.STERADIAN.)
SOLID_ANGLE_UNIT()
);
#18014=SHAPE_DEFINITION_REPRESENTATION(#18033,#18073);
#18033=PRODUCT_DEFINITION_SHAPE('',$,#18093);
#18073=SHAPE_REPRESENTATION('',(#10013),#17990);
#18089=PRODUCT_DEFINITION_CONTEXT('part definition',#18148,'design');
#18093=PRODUCT_DEFINITION('Right Upright','Right Upright',#18112,#18089);
#18112=PRODUCT_DEFINITION_FORMATION('',$,#18153);
#18148=APPLICATION_CONTEXT(
'Core Data for Automotive Mechanical Design Process');
#18149=PRODUCT_CONTEXT('part definition',#18148,'mechanical');
#18153=PRODUCT('Right Upright','Right Upright',$,(#18149));
#18170=PRESENTATION_STYLE_ASSIGNMENT((#18174));
#18174=SURFACE_STYLE_USAGE(.BOTH.,#18178);
#18178=SURFACE_SIDE_STYLE('',(#18182));
#18182=SURFACE_STYLE_FILL_AREA(#18186);
#18186=FILL_AREA_STYLE('Opaque(227,224,212)',(#18190));
#18190=FILL_AREA_STYLE_COLOUR('Opaque(227,224,212)',#18194);
#18194=COLOUR_RGB('Opaque(227,224,212)',0.890196078431372,0.87843137254902,
0.831372549019608);
ENDSEC;
END-ISO-10303-21;
